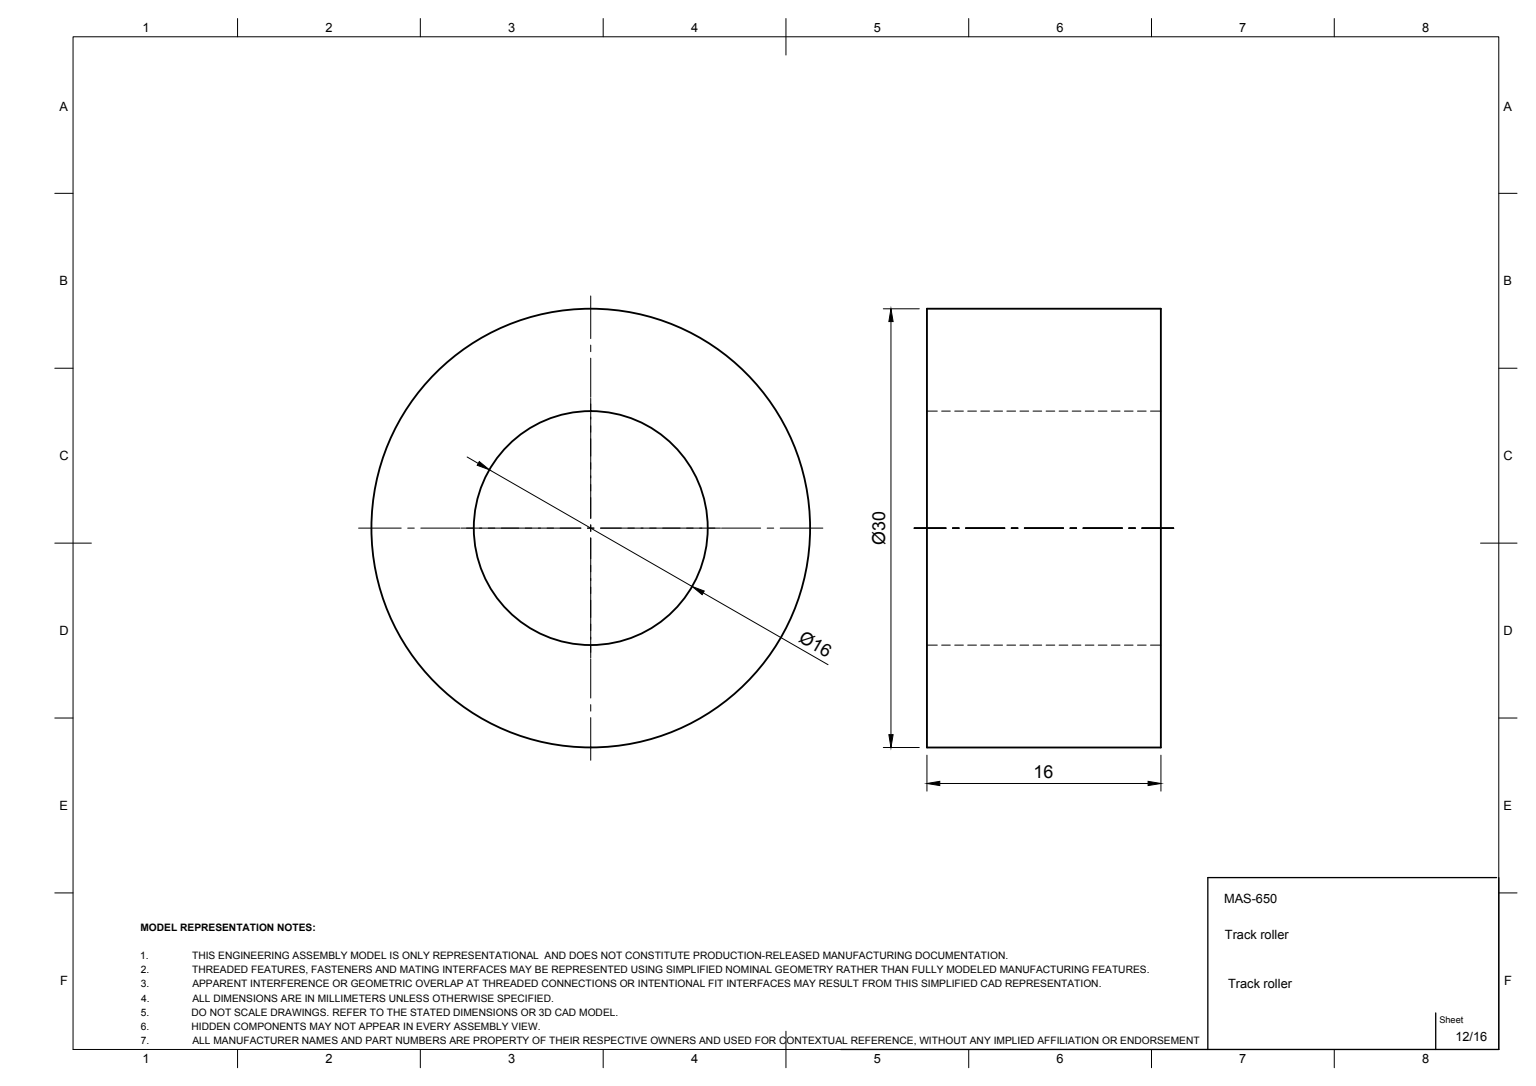
ISO-10303-21;
HEADER;
/* Generated by software containing ST-Developer
 * from STEP Tools, Inc. (www.steptools.com) 
 */

FILE_DESCRIPTION(
/* description */ ('Independent manual traversing gantry with native reusable aluminum pr
ofiles,180mm captured carriage travel, four bronze-bushed rollers, lin
ked ideal rolling motion, bonded acetal lateral guides, positive welde
d end stops and fully retained axle stacks. Editable native profile cu
t lengths220/400mm. Tool attachments viaM6 bridge-plate taps; mounted 
tool outside assembly. Welds, anchors, adhesives, fits, traction, load
/speed/structural/life ratings unassigned.'),
/* implementation_level */ '2;1');

FILE_NAME(
/* name */ 'Track roller.step',
/* time_stamp */ '2026-11-09T20:04:38-08:00',
/* author */ (''),
/* organization */ (''),
/* preprocessor_version */ 'ST-DEVELOPER v20.2',
/* originating_system */ 'Autodesk Translation Framework v15.17.0.0',
/* authorisation */ '');

FILE_SCHEMA (('AUTOMOTIVE_DESIGN { 1 0 10303 214 3 1 1 }'));
ENDSEC;

DATA;
#10=MECHANICAL_DESIGN_GEOMETRIC_PRESENTATION_REPRESENTATION('',(#480),#13231);
#448=SHAPE_REPRESENTATION_RELATIONSHIP('SRR','None',#13337,#464);
#464=ADVANCED_BREP_SHAPE_REPRESENTATION('',(#496),#13224);
#480=STYLED_ITEM('',(#13425),#496);
#496=MANIFOLD_SOLID_BREP('Body1',#4160);
#539=FACE_BOUND('',#1079,.T.);
#540=FACE_BOUND('',#1081,.T.);
#614=PLANE('',#4611);
#615=PLANE('',#4612);
#819=FACE_OUTER_BOUND('',#1076,.T.);
#820=FACE_OUTER_BOUND('',#1077,.T.);
#821=FACE_OUTER_BOUND('',#1078,.T.);
#822=FACE_OUTER_BOUND('',#1080,.T.);
#1076=EDGE_LOOP('',(#3690,#3691,#3692,#3693));
#1077=EDGE_LOOP('',(#3694,#3695,#3696,#3697));
#1078=EDGE_LOOP('',(#3698));
#1079=EDGE_LOOP('',(#3699));
#1080=EDGE_LOOP('',(#3700));
#1081=EDGE_LOOP('',(#3701));
#1364=LINE('',#13012,#1626);
#1365=LINE('',#13018,#1627);
#1626=VECTOR('',#5501,8.);
#1627=VECTOR('',#5508,15.);
#1720=CIRCLE('',#4606,8.);
#1721=CIRCLE('',#4607,8.);
#1722=CIRCLE('',#4609,15.);
#1723=CIRCLE('',#4610,15.);
#2088=VERTEX_POINT('',#13009);
#2089=VERTEX_POINT('',#13011);
#2090=VERTEX_POINT('',#13015);
#2091=VERTEX_POINT('',#13017);
#2628=EDGE_CURVE('',#2088,#2088,#1720,.T.);
#2629=EDGE_CURVE('',#2088,#2089,#1364,.T.);
#2630=EDGE_CURVE('',#2089,#2089,#1721,.T.);
#2631=EDGE_CURVE('',#2090,#2090,#1722,.T.);
#2632=EDGE_CURVE('',#2090,#2091,#1365,.T.);
#2633=EDGE_CURVE('',#2091,#2091,#1723,.T.);
#3690=ORIENTED_EDGE('',*,*,#2628,.F.);
#3691=ORIENTED_EDGE('',*,*,#2629,.T.);
#3692=ORIENTED_EDGE('',*,*,#2630,.T.);
#3693=ORIENTED_EDGE('',*,*,#2629,.F.);
#3694=ORIENTED_EDGE('',*,*,#2631,.F.);
#3695=ORIENTED_EDGE('',*,*,#2632,.T.);
#3696=ORIENTED_EDGE('',*,*,#2633,.T.);
#3697=ORIENTED_EDGE('',*,*,#2632,.F.);
#3698=ORIENTED_EDGE('',*,*,#2631,.T.);
#3699=ORIENTED_EDGE('',*,*,#2628,.T.);
#3700=ORIENTED_EDGE('',*,*,#2633,.F.);
#3701=ORIENTED_EDGE('',*,*,#2630,.F.);
#3914=CYLINDRICAL_SURFACE('',#4605,8.);
#3915=CYLINDRICAL_SURFACE('',#4608,15.);
#4116=ADVANCED_FACE('',(#819),#3914,.F.);
#4117=ADVANCED_FACE('',(#820),#3915,.T.);
#4118=ADVANCED_FACE('',(#821,#539),#614,.T.);
#4119=ADVANCED_FACE('',(#822,#540),#615,.F.);
#4160=CLOSED_SHELL('',(#4116,#4117,#4118,#4119));
#4604=AXIS2_PLACEMENT_3D('',#13007,#5495,#5496);
#4605=AXIS2_PLACEMENT_3D('',#13008,#5497,#5498);
#4606=AXIS2_PLACEMENT_3D('',#13010,#5499,#5500);
#4607=AXIS2_PLACEMENT_3D('',#13013,#5502,#5503);
#4608=AXIS2_PLACEMENT_3D('',#13014,#5504,#5505);
#4609=AXIS2_PLACEMENT_3D('',#13016,#5506,#5507);
#4610=AXIS2_PLACEMENT_3D('',#13019,#5509,#5510);
#4611=AXIS2_PLACEMENT_3D('',#13020,#5511,#5512);
#4612=AXIS2_PLACEMENT_3D('',#13021,#5513,#5514);
#5495=DIRECTION('axis',(0.,0.,1.));
#5496=DIRECTION('refdir',(1.,0.,0.));
#5497=DIRECTION('center_axis',(0.,0.,1.));
#5498=DIRECTION('ref_axis',(1.,0.,0.));
#5499=DIRECTION('center_axis',(0.,0.,-1.));
#5500=DIRECTION('ref_axis',(1.,0.,0.));
#5501=DIRECTION('',(0.,0.,-1.));
#5502=DIRECTION('center_axis',(0.,0.,-1.));
#5503=DIRECTION('ref_axis',(1.,0.,0.));
#5504=DIRECTION('center_axis',(0.,0.,1.));
#5505=DIRECTION('ref_axis',(1.,0.,0.));
#5506=DIRECTION('center_axis',(0.,0.,1.));
#5507=DIRECTION('ref_axis',(1.,0.,0.));
#5508=DIRECTION('',(0.,0.,-1.));
#5509=DIRECTION('center_axis',(0.,0.,1.));
#5510=DIRECTION('ref_axis',(1.,0.,0.));
#5511=DIRECTION('center_axis',(0.,0.,1.));
#5512=DIRECTION('ref_axis',(1.,0.,0.));
#5513=DIRECTION('center_axis',(0.,0.,1.));
#5514=DIRECTION('ref_axis',(1.,0.,0.));
#13007=CARTESIAN_POINT('',(0.,0.,0.));
#13008=CARTESIAN_POINT('Origin',(0.,0.,0.));
#13009=CARTESIAN_POINT('',(-8.,-9.79717439317883E-16,16.));
#13010=CARTESIAN_POINT('Origin',(0.,0.,16.));
#13011=CARTESIAN_POINT('',(-8.,-9.79717439317883E-16,0.));
#13012=CARTESIAN_POINT('',(-8.,-9.79717439317883E-16,0.));
#13013=CARTESIAN_POINT('Origin',(0.,0.,0.));
#13014=CARTESIAN_POINT('Origin',(0.,0.,0.));
#13015=CARTESIAN_POINT('',(-15.,-1.83697019872103E-15,16.));
#13016=CARTESIAN_POINT('Origin',(0.,0.,16.));
#13017=CARTESIAN_POINT('',(-15.,-1.83697019872103E-15,0.));
#13018=CARTESIAN_POINT('',(-15.,-1.83697019872103E-15,0.));
#13019=CARTESIAN_POINT('Origin',(0.,0.,0.));
#13020=CARTESIAN_POINT('Origin',(0.,0.,16.));
#13021=CARTESIAN_POINT('Origin',(0.,0.,0.));
#13206=UNCERTAINTY_MEASURE_WITH_UNIT(LENGTH_MEASURE(0.01),#13232,
'DISTANCE_ACCURACY_VALUE',
'Maximum model space distance between geometric entities at asserted c
onnectivities');
#13213=UNCERTAINTY_MEASURE_WITH_UNIT(LENGTH_MEASURE(0.01),#13232,
'DISTANCE_ACCURACY_VALUE',
'Maximum model space distance between geometric entities at asserted c
onnectivities');
#13224=(
GEOMETRIC_REPRESENTATION_CONTEXT(3)
GLOBAL_UNCERTAINTY_ASSIGNED_CONTEXT((#13206))
GLOBAL_UNIT_ASSIGNED_CONTEXT((#13232,#13234,#13235))
REPRESENTATION_CONTEXT('','3D')
);
#13231=(
GEOMETRIC_REPRESENTATION_CONTEXT(3)
GLOBAL_UNCERTAINTY_ASSIGNED_CONTEXT((#13213))
GLOBAL_UNIT_ASSIGNED_CONTEXT((#13232,#13234,#13235))
REPRESENTATION_CONTEXT('','3D')
);
#13232=(
LENGTH_UNIT()
NAMED_UNIT(*)
SI_UNIT(.MILLI.,.METRE.)
);
#13234=(
NAMED_UNIT(*)
PLANE_ANGLE_UNIT()
SI_UNIT($,.RADIAN.)
);
#13235=(
NAMED_UNIT(*)
SI_UNIT($,.STERADIAN.)
SOLID_ANGLE_UNIT()
);
#13246=SHAPE_DEFINITION_REPRESENTATION(#13263,#13337);
#13263=PRODUCT_DEFINITION_SHAPE('',$,#13355);
#13337=SHAPE_REPRESENTATION('',(#4604),#13224);
#13344=PRODUCT_DEFINITION_CONTEXT('part definition',#13397,'design');
#13355=PRODUCT_DEFINITION('Track roller','Track roller',#13372,#13344);
#13372=PRODUCT_DEFINITION_FORMATION('',$,#13409);
#13397=APPLICATION_CONTEXT(
'Core Data for Automotive Mechanical Design Process');
#13398=PRODUCT_CONTEXT('part definition',#13397,'mechanical');
#13409=PRODUCT('Track roller','Track roller',$,(#13398));
#13425=PRESENTATION_STYLE_ASSIGNMENT((#13439));
#13439=SURFACE_STYLE_USAGE(.BOTH.,#13453);
#13453=SURFACE_SIDE_STYLE('',(#13467));
#13467=SURFACE_STYLE_FILL_AREA(#13481);
#13481=FILL_AREA_STYLE('Sky blue',(#13495));
#13495=FILL_AREA_STYLE_COLOUR('Sky blue',#13509);
#13509=COLOUR_RGB('Sky blue',0.317647058823529,0.686274509803922,0.890196078431372);
ENDSEC;
END-ISO-10303-21;
